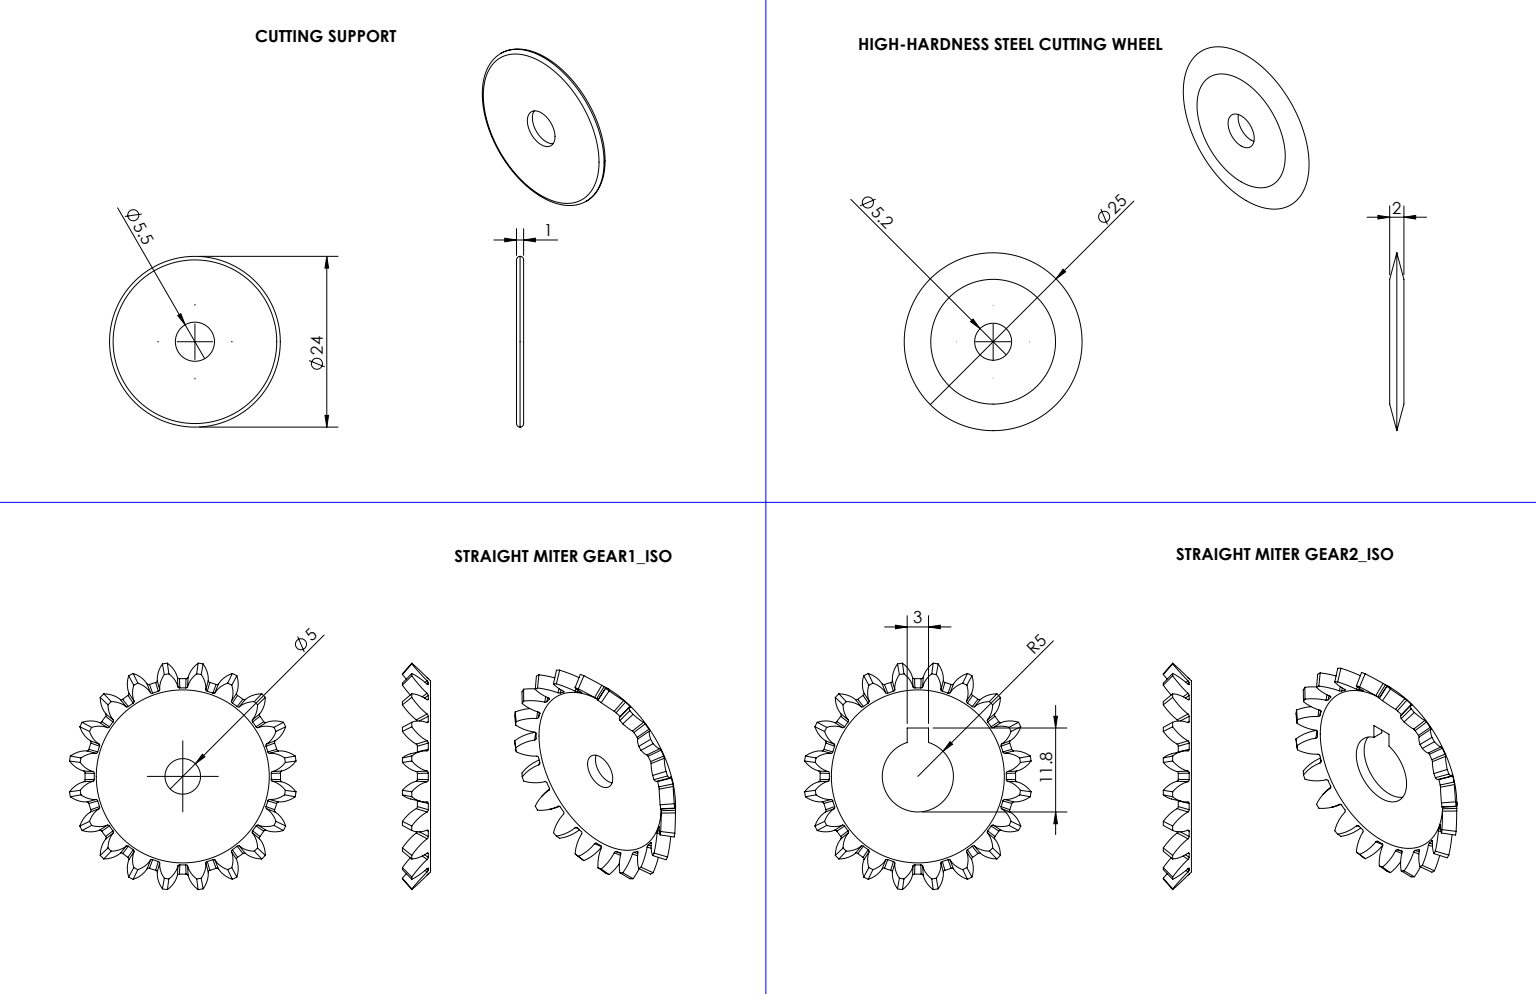
ISO-10303-21;
HEADER;
FILE_DESCRIPTION (('STEP AP214'),
    '1' );
FILE_NAME ('High-Hardness Steel Cutting Wheel.step',
    '2026-09-24T10:15:42',
    ( '' ),
    ( '' ),
    'SwSTEP 2.0',
    'SolidWorks 2026',
    '' );
FILE_SCHEMA (( 'AUTOMOTIVE_DESIGN' ));
ENDSEC;

DATA;
#92=FACE_BOUND ( 'NONE', #18498, .T. ) ;
#132=ORIENTED_EDGE ( 'NONE', *, *, #4909, .F. ) ;
#187=EDGE_LOOP ( 'NONE', ( #15081, #15539 ) ) ;
#218=SURFACE_SIDE_STYLE ('',( #5937 ) ) ;
#256=VERTEX_POINT ( 'NONE', #16289 ) ;
#279=ORIENTED_EDGE ( 'NONE', *, *, #2294, .T. ) ;
#396=MECHANICAL_DESIGN_GEOMETRIC_PRESENTATION_REPRESENTATION('',(#14763),#11087);
#455=PRODUCT_DEFINITION_CONTEXT ( 'detailed design', #9607, 'design' ) ;
#466=AXIS2_PLACEMENT_3D ( 'NONE', #18241, #2269, #18054 ) ;
#565=DIRECTION ( 'NONE',  ( -0.000000000000000000, 1.000000000000000000, -0.000000000000000000 ) ) ;
#601=ADVANCED_FACE ( 'NONE', ( #10334 ), #6040, .F. ) ;
#657=ORIENTED_EDGE ( 'NONE', *, *, #5467, .T. ) ;
#781=DIRECTION ( 'NONE',  ( 0.000000000000000000, -1.000000000000000000, 0.000000000000000000 ) ) ;
#795=EDGE_LOOP ( 'NONE', ( #16035, #279, #1272, #10918 ) ) ;
#851=ADVANCED_FACE ( 'NONE', ( #17477, #10119 ), #8682, .F. ) ;
#884=EDGE_LOOP ( 'NONE', ( #132, #11644, #15801, #8362 ) ) ;
#997=ORIENTED_EDGE ( 'NONE', *, *, #13718, .T. ) ;
#1073=EDGE_CURVE ( 'NONE', #15587, #15699, #16006, .T. ) ;
#1102=( GEOMETRIC_REPRESENTATION_CONTEXT ( 3 ) GLOBAL_UNCERTAINTY_ASSIGNED_CONTEXT ( ( #11702 ) ) GLOBAL_UNIT_ASSIGNED_CONTEXT ( ( #6049, #7298, #13114 ) ) REPRESENTATION_CONTEXT ( 'NONE', 'WORKASPACE' ) );
#1175=DIRECTION ( 'NONE',  ( 1.540743955509788340E-33, 1.000000000000000000, 2.533398541561209262E-17 ) ) ;
#1245=DIRECTION ( 'NONE',  ( 0.000000000000000000, 0.000000000000000000, 1.000000000000000000 ) ) ;
#1272=ORIENTED_EDGE ( 'NONE', *, *, #5435, .F. ) ;
#1327=CARTESIAN_POINT ( 'NONE',  ( 1.321128355694181398E-14, -7.013167318348350499, 25.01316734529530095 ) ) ;
#1414=PRODUCT ( 'High-Hardness Steel Cutting Wheel', 'High-Hardness Steel Cutting Wheel', '', ( #12280 ) ) ;
#1442=EDGE_LOOP ( 'NONE', ( #18668, #4195, #17241, #11960 ) ) ;
#1444=DIRECTION ( 'NONE',  ( 1.540743955509788340E-33, 1.000000000000000000, 2.533398541561209262E-17 ) ) ;
#1471=PRODUCT_DEFINITION ( 'UNKNOWN', '', #4710, #455 ) ;
#1479=EDGE_CURVE ( 'NONE', #15020, #256, #1980, .T. ) ;
#1562=AXIS2_PLACEMENT_3D ( 'NONE', #11635, #5692, #17463 ) ;
#1662=FACE_OUTER_BOUND ( 'NONE', #1442, .T. ) ;
#1671=VECTOR ( 'NONE', #15487, 1000.000000000000114 ) ;
#1803=ORIENTED_EDGE ( 'NONE', *, *, #4909, .T. ) ;
#1812=AXIS2_PLACEMENT_3D ( 'NONE', #15485, #781, #18442 ) ;
#1888=DIRECTION ( 'NONE',  ( -1.540743955509788340E-33, -1.000000000000000000, -2.533398541561209262E-17 ) ) ;
#1965=CARTESIAN_POINT ( 'NONE',  ( 1.451356985208877954E-14, -9.013167318348349610, 16.24521815286417947 ) ) ;
#1980=LINE ( 'NONE', #7820, #2247 ) ;
#2030=AXIS2_PLACEMENT_3D ( 'NONE', #15716, #11248, #17249 ) ;
#2049=AXIS2_PLACEMENT_3D ( 'NONE', #17593, #1444, #9087 ) ;
#2084=CONICAL_SURFACE ( 'NONE', #18539, 12.50000000000000355, 1.308996938995747428 ) ;
#2229=CARTESIAN_POINT ( 'NONE',  ( 1.321128355694181398E-14, -7.013167318348350499, 25.01316734529530095 ) ) ;
#2236=SURFACE_STYLE_FILL_AREA ( #9686 ) ;
#2247=VECTOR ( 'NONE', #6907, 1000.000000000000114 ) ;
#2269=DIRECTION ( 'NONE',  ( 1.540743955509788340E-33, 1.000000000000000000, 2.533398541561209262E-17 ) ) ;
#2294=EDGE_CURVE ( 'NONE', #12560, #15587, #14969, .T. ) ;
#2327=( NAMED_UNIT ( * ) PLANE_ANGLE_UNIT ( ) SI_UNIT ( $, .RADIAN. ) );
#2395=ORIENTED_EDGE ( 'NONE', *, *, #9782, .F. ) ;
#2464=EDGE_LOOP ( 'NONE', ( #11141, #1803, #13657, #3611 ) ) ;
#2532=DIRECTION ( 'NONE',  ( 0.000000000000000000, -0.2588190451025214611, -0.9659258262890679791 ) ) ;
#2742=DIRECTION ( 'NONE',  ( 0.000000000000000000, -2.533398541561209262E-17, 1.000000000000000000 ) ) ;
#2746=DIRECTION ( 'NONE',  ( 0.000000000000000000, -2.533398541561209262E-17, 1.000000000000000000 ) ) ;
#2869=DIRECTION ( 'NONE',  ( -0.000000000000000000, 1.000000000000000000, -0.000000000000000000 ) ) ;
#2879=VECTOR ( 'NONE', #2532, 1000.000000000000114 ) ;
#2951=CARTESIAN_POINT ( 'NONE',  ( 1.321128355694181398E-14, -8.013167318348353163, 12.51316734529529562 ) ) ;
#3058=PRESENTATION_STYLE_ASSIGNMENT (( #4615 ) ) ;
#3059=DIRECTION ( 'NONE',  ( 0.000000000000000000, 0.000000000000000000, 1.000000000000000000 ) ) ;
#3319=ORIENTED_EDGE ( 'NONE', *, *, #1073, .F. ) ;
#3343=VERTEX_POINT ( 'NONE', #18411 ) ;
#3495=EDGE_LOOP ( 'NONE', ( #9973, #17749 ) ) ;
#3611=ORIENTED_EDGE ( 'NONE', *, *, #1479, .F. ) ;
#3694=FACE_OUTER_BOUND ( 'NONE', #2464, .T. ) ;
#3833=LINE ( 'NONE', #9659, #1671 ) ;
#3858=( NAMED_UNIT ( * ) PLANE_ANGLE_UNIT ( ) SI_UNIT ( $, .RADIAN. ) );
#4195=ORIENTED_EDGE ( 'NONE', *, *, #5467, .F. ) ;
#4383=DIRECTION ( 'NONE',  ( 1.540743955509788340E-33, 1.000000000000000000, 2.533398541561209262E-17 ) ) ;
#4568=CIRCLE ( 'NONE', #13723, 12.50000000000000355 ) ;
#4615=SURFACE_STYLE_USAGE ( .BOTH. , #218 ) ;
#4710=PRODUCT_DEFINITION_FORMATION_WITH_SPECIFIED_SOURCE ( 'ANY', '', #1414, .NOT_KNOWN. ) ;
#4808=AXIS2_PLACEMENT_3D ( 'NONE', #7609, #12190, #7799 ) ;
#4909=EDGE_CURVE ( 'NONE', #18033, #5504, #7459, .T. ) ;
#5081=MECHANICAL_DESIGN_GEOMETRIC_PRESENTATION_REPRESENTATION('',(#16981),#1102);
#5195=SURFACE_SIDE_STYLE ('',( #2236 ) ) ;
#5244=EDGE_CURVE ( 'NONE', #12234, #3343, #18505, .T. ) ;
#5407=CARTESIAN_POINT ( 'NONE',  ( 1.104287921197080512E-14, -7.013167318348350499, 22.41316734529519650 ) ) ;
#5435=EDGE_CURVE ( 'NONE', #15699, #15587, #8163, .T. ) ;
#5467=EDGE_CURVE ( 'NONE', #3343, #12234, #10605, .T. ) ;
#5504=VERTEX_POINT ( 'NONE', #2951 ) ;
#5532=CARTESIAN_POINT ( 'NONE',  ( 1.104287921197080512E-14, -7.013167318348350499, 22.41316734529519650 ) ) ;
#5692=DIRECTION ( 'NONE',  ( -1.540743955509788340E-33, -1.000000000000000000, -2.533398541561209262E-17 ) ) ;
#5820=AXIS2_PLACEMENT_3D ( 'NONE', #15005, #7668, #11955 ) ;
#5937=SURFACE_STYLE_FILL_AREA ( #10440 ) ;
#5991=DIRECTION ( 'NONE',  ( 0.000000000000000000, 0.000000000000000000, 1.000000000000000000 ) ) ;
#6040=CYLINDRICAL_SURFACE ( 'NONE', #13619, 2.600000000000092015 ) ;
#6049=( LENGTH_UNIT ( ) NAMED_UNIT ( * ) SI_UNIT ( .MILLI., .METRE. ) );
#6129=CYLINDRICAL_SURFACE ( 'NONE', #5820, 2.600000000000092015 ) ;
#6330=DIRECTION ( 'NONE',  ( 0.000000000000000000, 0.000000000000000000, -1.000000000000000000 ) ) ;
#6514=ORIENTED_EDGE ( 'NONE', *, *, #17078, .F. ) ;
#6622=COLOUR_RGB ( '', 0.08235294, 0.09019608, 0.10196078) ;
#6708=ORIENTED_EDGE ( 'NONE', *, *, #18094, .T. ) ;
#6739=SHAPE_DEFINITION_REPRESENTATION ( #17767, #13515 ) ;
#6907=DIRECTION ( 'NONE',  ( 0.000000000000000000, 0.2588190451025206285, 0.9659258262890683122 ) ) ;
#6917=( LENGTH_UNIT ( ) NAMED_UNIT ( * ) SI_UNIT ( .MILLI., .METRE. ) );
#7015=DIRECTION ( 'NONE',  ( 0.000000000000000000, 0.000000000000000000, 1.000000000000000000 ) ) ;
#7174=DIRECTION ( 'NONE',  ( 1.540743955509788340E-33, 1.000000000000000000, 2.533398541561209262E-17 ) ) ;
#7248=DIRECTION ( 'NONE',  ( 0.000000000000000000, -1.000000000000000000, 0.000000000000000000 ) ) ;
#7249=CLOSED_SHELL ( 'NONE', ( #13576, #7332, #601, #8241, #851, #12848, #16673, #11406 ) ) ;
#7298=( NAMED_UNIT ( * ) PLANE_ANGLE_UNIT ( ) SI_UNIT ( $, .RADIAN. ) );
#7332=ADVANCED_FACE ( 'NONE', ( #15316 ), #12653, .T. ) ;
#7459=LINE ( 'NONE', #11846, #8088 ) ;
#7463=CARTESIAN_POINT ( 'NONE',  ( 1.321128355694181398E-14, -9.013167318348349610, 25.01316734529530095 ) ) ;
#7609=CARTESIAN_POINT ( 'NONE',  ( 1.321128355694181398E-14, -7.013167318348350499, 25.01316734529530095 ) ) ;
#7668=DIRECTION ( 'NONE',  ( -1.540743955509788340E-33, -1.000000000000000000, -2.533398541561209262E-17 ) ) ;
#7752=CONICAL_SURFACE ( 'NONE', #18696, 12.50000000000000355, 1.308996938995747428 ) ;
#7799=DIRECTION ( 'NONE',  ( 0.000000000000000000, 0.000000000000000000, -1.000000000000000000 ) ) ;
#7820=CARTESIAN_POINT ( 'NONE',  ( 1.321128355694181398E-14, -8.013167318348349610, 37.51316734529530805 ) ) ;
#7832=CARTESIAN_POINT ( 'NONE',  ( 1.321128355694181398E-14, -8.013167318348349610, 25.01316734529530095 ) ) ;
#7885=CARTESIAN_POINT ( 'NONE',  ( 1.136128737974912818E-14, -7.013167318348350499, 27.61316734529538053 ) ) ;
#7966=EDGE_CURVE ( 'NONE', #3343, #5504, #15454, .T. ) ;
#8062=DIRECTION ( 'NONE',  ( 0.000000000000000000, 0.000000000000000000, 1.000000000000000000 ) ) ;
#8083=CARTESIAN_POINT ( 'NONE',  ( 1.451356985208878270E-14, -7.013167318348350499, 33.78111653772643308 ) ) ;
#8088=VECTOR ( 'NONE', #17577, 1000.000000000000114 ) ;
#8163=CIRCLE ( 'NONE', #18823, 2.600000000000092015 ) ;
#8241=ADVANCED_FACE ( 'NONE', ( #8593, #92 ), #17685, .T. ) ;
#8265=( LENGTH_UNIT ( ) NAMED_UNIT ( * ) SI_UNIT ( .MILLI., .METRE. ) );
#8362=ORIENTED_EDGE ( 'NONE', *, *, #17496, .T. ) ;
#8375=EDGE_LOOP ( 'NONE', ( #16741, #10834, #997, #3319 ) ) ;
#8466=DIRECTION ( 'NONE',  ( -1.540743955509788340E-33, -1.000000000000000000, -2.533398541561209262E-17 ) ) ;
#8516=CARTESIAN_POINT ( 'NONE',  ( 1.104287921197080512E-14, -9.013167318348349610, 25.01316734529528674 ) ) ;
#8593=FACE_OUTER_BOUND ( 'NONE', #13210, .T. ) ;
#8629=APPLICATION_CONTEXT ( 'automotive_design' ) ;
#8659=ORIENTED_EDGE ( 'NONE', *, *, #7966, .F. ) ;
#8682=PLANE ( 'NONE',  #14026 ) ;
#9004=ADVANCED_BREP_SHAPE_REPRESENTATION ( '', ( #10342, #2030 ), #13001 ) ;
#9007=SHAPE_REPRESENTATION_RELATIONSHIP ( 'NONE' , 'NONE' ,  #13515, #9004 ) ;
#9087=DIRECTION ( 'NONE',  ( 0.000000000000000000, 0.000000000000000000, 1.000000000000000000 ) ) ;
#9132=CARTESIAN_POINT ( 'NONE',  ( 1.321128355694181398E-14, -9.013167318348349610, 33.78111653772642597 ) ) ;
#9178=FACE_OUTER_BOUND ( 'NONE', #8375, .T. ) ;
#9607=APPLICATION_CONTEXT ( 'automotive_design' ) ;
#9659=CARTESIAN_POINT ( 'NONE',  ( 1.428504764830155575E-14, -7.013167318348350499, 33.78111653772643308 ) ) ;
#9686=FILL_AREA_STYLE ('',( #15865 ) ) ;
#9782=EDGE_CURVE ( 'NONE', #12560, #18215, #17894, .T. ) ;
#9926=DIRECTION ( 'NONE',  ( 1.540743955509788340E-33, 1.000000000000000000, 2.533398541561209262E-17 ) ) ;
#9973=ORIENTED_EDGE ( 'NONE', *, *, #17326, .T. ) ;
#10034=CIRCLE ( 'NONE', #1812, 12.50000000000000355 ) ;
#10119=FACE_BOUND ( 'NONE', #187, .T. ) ;
#10334=FACE_OUTER_BOUND ( 'NONE', #795, .T. ) ;
#10342=MANIFOLD_SOLID_BREP ( 'Chamfer2', #7249 ) ;
#10368=UNCERTAINTY_MEASURE_WITH_UNIT (LENGTH_MEASURE( 1.000000000000000082E-05 ), #6917, 'distance_accuracy_value', 'NONE');
#10440=FILL_AREA_STYLE ('',( #17417 ) ) ;
#10531=ORIENTED_EDGE ( 'NONE', *, *, #11357, .F. ) ;
#10605=CIRCLE ( 'NONE', #2049, 8.767949192431130356 ) ;
#10746=DIRECTION ( 'NONE',  ( 0.000000000000000000, 0.000000000000000000, -1.000000000000000000 ) ) ;
#10834=ORIENTED_EDGE ( 'NONE', *, *, #9782, .T. ) ;
#10918=ORIENTED_EDGE ( 'NONE', *, *, #13718, .F. ) ;
#10988=AXIS2_PLACEMENT_3D ( 'NONE', #7463, #17878, #14905 ) ;
#11087=( GEOMETRIC_REPRESENTATION_CONTEXT ( 3 ) GLOBAL_UNCERTAINTY_ASSIGNED_CONTEXT ( ( #12635 ) ) GLOBAL_UNIT_ASSIGNED_CONTEXT ( ( #8265, #2327, #13889 ) ) REPRESENTATION_CONTEXT ( 'NONE', 'WORKASPACE' ) );
#11141=ORIENTED_EDGE ( 'NONE', *, *, #12931, .F. ) ;
#11248=DIRECTION ( 'NONE',  ( 0.000000000000000000, 0.000000000000000000, 1.000000000000000000 ) ) ;
#11263=CARTESIAN_POINT ( 'NONE',  ( 1.321128355694181398E-14, -7.013167318348350499, 16.24521815286417237 ) ) ;
#11357=EDGE_CURVE ( 'NONE', #18215, #12560, #15963, .T. ) ;
#11406=ADVANCED_FACE ( 'NONE', ( #13206 ), #7752, .T. ) ;
#11475=CARTESIAN_POINT ( 'NONE',  ( 1.104287921197080512E-14, -7.013167318348350499, 25.01316734529528674 ) ) ;
#11572=SURFACE_STYLE_USAGE ( .BOTH. , #5195 ) ;
#11600=ORIENTED_EDGE ( 'NONE', *, *, #5244, .T. ) ;
#11635=CARTESIAN_POINT ( 'NONE',  ( 1.321128355694181398E-14, -9.013167318348349610, 25.01316734529530095 ) ) ;
#11644=ORIENTED_EDGE ( 'NONE', *, *, #17326, .F. ) ;
#11702=UNCERTAINTY_MEASURE_WITH_UNIT (LENGTH_MEASURE( 1.000000000000000082E-05 ), #6049, 'distance_accuracy_value', 'NONE');
#11741=VECTOR ( 'NONE', #1888, 1000.000000000000000 ) ;
#11846=CARTESIAN_POINT ( 'NONE',  ( 1.474209205587600649E-14, -8.013167318348349610, 12.51316734529529562 ) ) ;
#11955=DIRECTION ( 'NONE',  ( 0.000000000000000000, 0.000000000000000000, -1.000000000000000000 ) ) ;
#11960=ORIENTED_EDGE ( 'NONE', *, *, #17496, .F. ) ;
#12190=DIRECTION ( 'NONE',  ( 0.000000000000000000, -1.000000000000000000, 0.000000000000000000 ) ) ;
#12234=VERTEX_POINT ( 'NONE', #8083 ) ;
#12280=PRODUCT_CONTEXT ( 'NONE', #8629, 'mechanical' ) ;
#12393=DIRECTION ( 'NONE',  ( 0.000000000000000000, 0.000000000000000000, 1.000000000000000000 ) ) ;
#12560=VERTEX_POINT ( 'NONE', #7885 ) ;
#12635=UNCERTAINTY_MEASURE_WITH_UNIT (LENGTH_MEASURE( 1.000000000000000082E-05 ), #8265, 'distance_accuracy_value', 'NONE');
#12653=CONICAL_SURFACE ( 'NONE', #13573, 8.767949192431130356, 1.308996938995746318 ) ;
#12793=CARTESIAN_POINT ( 'NONE',  ( 1.321128355694181398E-14, -9.013167318348349610, 25.01316734529530095 ) ) ;
#12848=ADVANCED_FACE ( 'NONE', ( #9178 ), #6129, .F. ) ;
#12931=EDGE_CURVE ( 'NONE', #18033, #15020, #15900, .T. ) ;
#13001=( GEOMETRIC_REPRESENTATION_CONTEXT ( 3 ) GLOBAL_UNCERTAINTY_ASSIGNED_CONTEXT ( ( #10368 ) ) GLOBAL_UNIT_ASSIGNED_CONTEXT ( ( #6917, #3858, #18565 ) ) REPRESENTATION_CONTEXT ( 'NONE', 'WORKASPACE' ) );
#13018=CARTESIAN_POINT ( 'NONE',  ( 1.321128355694181398E-14, -8.013167318348349610, 25.01316734529530095 ) ) ;
#13114=( NAMED_UNIT ( * ) SI_UNIT ( $, .STERADIAN. ) SOLID_ANGLE_UNIT ( ) );
#13206=FACE_OUTER_BOUND ( 'NONE', #884, .T. ) ;
#13210=EDGE_LOOP ( 'NONE', ( #657, #11600 ) ) ;
#13353=CARTESIAN_POINT ( 'NONE',  ( 1.321128355694181398E-14, -8.013167318348353163, 25.01316734529530095 ) ) ;
#13515=SHAPE_REPRESENTATION ( 'High-Hardness Steel Cutting Wheel', ( #2030 ), #13001 ) ;
#13573=AXIS2_PLACEMENT_3D ( 'NONE', #2229, #13609, #10746 ) ;
#13576=ADVANCED_FACE ( 'NONE', ( #3694 ), #2084, .T. ) ;
#13609=DIRECTION ( 'NONE',  ( 0.000000000000000000, -1.000000000000000000, 0.000000000000000000 ) ) ;
#13619=AXIS2_PLACEMENT_3D ( 'NONE', #16365, #16265, #6330 ) ;
#13657=ORIENTED_EDGE ( 'NONE', *, *, #17078, .T. ) ;
#13718=EDGE_CURVE ( 'NONE', #18215, #15699, #14381, .T. ) ;
#13723=AXIS2_PLACEMENT_3D ( 'NONE', #13353, #7248, #5991 ) ;
#13889=( NAMED_UNIT ( * ) SI_UNIT ( $, .STERADIAN. ) SOLID_ANGLE_UNIT ( ) );
#13970=CARTESIAN_POINT ( 'NONE',  ( 1.136128737974912818E-14, -9.013167318348349610, 27.61316734529538053 ) ) ;
#14026=AXIS2_PLACEMENT_3D ( 'NONE', #12793, #4383, #2742 ) ;
#14058=DIRECTION ( 'NONE',  ( 0.000000000000000000, 0.000000000000000000, 1.000000000000000000 ) ) ;
#14274=CARTESIAN_POINT ( 'NONE',  ( 1.104287921197080512E-14, -7.013167318348350499, 25.01316734529528674 ) ) ;
#14341=DIRECTION ( 'NONE',  ( 1.540743955509788340E-33, 1.000000000000000000, 2.533398541561209262E-17 ) ) ;
#14381=LINE ( 'NONE', #5407, #16116 ) ;
#14504=AXIS2_PLACEMENT_3D ( 'NONE', #11475, #7174, #14058 ) ;
#14763=STYLED_ITEM ( 'NONE', ( #17292 ), #10342 ) ;
#14905=DIRECTION ( 'NONE',  ( 0.000000000000000000, 0.000000000000000000, 1.000000000000000000 ) ) ;
#14969=LINE ( 'NONE', #17849, #11741 ) ;
#15005=CARTESIAN_POINT ( 'NONE',  ( 1.104287921197080512E-14, -7.013167318348350499, 25.01316734529528674 ) ) ;
#15020=VERTEX_POINT ( 'NONE', #9132 ) ;
#15081=ORIENTED_EDGE ( 'NONE', *, *, #5435, .T. ) ;
#15224=DIRECTION ( 'NONE',  ( 1.540743955509788340E-33, 1.000000000000000000, 2.533398541561209262E-17 ) ) ;
#15307=CARTESIAN_POINT ( 'NONE',  ( 1.321128355694181398E-14, -7.013167318348350499, 25.01316734529530095 ) ) ;
#15316=FACE_OUTER_BOUND ( 'NONE', #16211, .T. ) ;
#15454=LINE ( 'NONE', #11263, #2879 ) ;
#15485=CARTESIAN_POINT ( 'NONE',  ( 1.321128355694181398E-14, -8.013167318348353163, 25.01316734529530095 ) ) ;
#15487=DIRECTION ( 'NONE',  ( 1.182917971378669349E-16, -0.2588190451025214611, 0.9659258262890679791 ) ) ;
#15539=ORIENTED_EDGE ( 'NONE', *, *, #1073, .T. ) ;
#15587=VERTEX_POINT ( 'NONE', #13970 ) ;
#15699=VERTEX_POINT ( 'NONE', #16160 ) ;
#15716=CARTESIAN_POINT ( 'NONE',  ( 0.000000000000000000, 0.000000000000000000, 0.000000000000000000 ) ) ;
#15801=ORIENTED_EDGE ( 'NONE', *, *, #1479, .T. ) ;
#15865=FILL_AREA_STYLE_COLOUR ( '', #16873 ) ;
#15900=CIRCLE ( 'NONE', #1562, 8.767949192431123251 ) ;
#15963=CIRCLE ( 'NONE', #18108, 2.600000000000092015 ) ;
#16006=CIRCLE ( 'NONE', #466, 2.600000000000092015 ) ;
#16035=ORIENTED_EDGE ( 'NONE', *, *, #11357, .T. ) ;
#16116=VECTOR ( 'NONE', #8466, 1000.000000000000000 ) ;
#16160=CARTESIAN_POINT ( 'NONE',  ( 1.104287921197080512E-14, -9.013167318348349610, 22.41316734529519650 ) ) ;
#16211=EDGE_LOOP ( 'NONE', ( #17374, #6708, #6514, #8659 ) ) ;
#16265=DIRECTION ( 'NONE',  ( -1.540743955509788340E-33, -1.000000000000000000, -2.533398541561209262E-17 ) ) ;
#16289=CARTESIAN_POINT ( 'NONE',  ( 1.474209205587600965E-14, -8.013167318348353163, 37.51316734529530805 ) ) ;
#16365=CARTESIAN_POINT ( 'NONE',  ( 1.104287921197080512E-14, -7.013167318348350499, 25.01316734529528674 ) ) ;
#16673=ADVANCED_FACE ( 'NONE', ( #1662 ), #18826, .T. ) ;
#16697=AXIS2_PLACEMENT_3D ( 'NONE', #15307, #15224, #8062 ) ;
#16741=ORIENTED_EDGE ( 'NONE', *, *, #2294, .F. ) ;
#16873=COLOUR_RGB ( '', 0.08235294, 0.09019608, 0.10196078) ;
#16981=STYLED_ITEM ( 'NONE', ( #3058 ), #9004 ) ;
#17078=EDGE_CURVE ( 'NONE', #5504, #256, #10034, .T. ) ;
#17241=ORIENTED_EDGE ( 'NONE', *, *, #7966, .T. ) ;
#17249=DIRECTION ( 'NONE',  ( 1.000000000000000000, 0.000000000000000000, 0.000000000000000000 ) ) ;
#17292=PRESENTATION_STYLE_ASSIGNMENT (( #11572 ) ) ;
#17326=EDGE_CURVE ( 'NONE', #15020, #18033, #17697, .T. ) ;
#17374=ORIENTED_EDGE ( 'NONE', *, *, #5244, .F. ) ;
#17417=FILL_AREA_STYLE_COLOUR ( '', #6622 ) ;
#17463=DIRECTION ( 'NONE',  ( 0.000000000000000000, 0.000000000000000000, 1.000000000000000000 ) ) ;
#17477=FACE_OUTER_BOUND ( 'NONE', #3495, .T. ) ;
#17496=EDGE_CURVE ( 'NONE', #256, #5504, #4568, .T. ) ;
#17577=DIRECTION ( 'NONE',  ( 1.182917971378669595E-16, 0.2588190451025206285, -0.9659258262890683122 ) ) ;
#17593=CARTESIAN_POINT ( 'NONE',  ( 1.321128355694181398E-14, -7.013167318348350499, 25.01316734529530095 ) ) ;
#17685=PLANE ( 'NONE',  #17870 ) ;
#17697=CIRCLE ( 'NONE', #10988, 8.767949192431123251 ) ;
#17749=ORIENTED_EDGE ( 'NONE', *, *, #12931, .T. ) ;
#17767=PRODUCT_DEFINITION_SHAPE ( 'NONE', 'NONE',  #1471 ) ;
#17849=CARTESIAN_POINT ( 'NONE',  ( 1.136128737974912818E-14, -7.013167318348350499, 27.61316734529538053 ) ) ;
#17870=AXIS2_PLACEMENT_3D ( 'NONE', #1327, #9926, #2746 ) ;
#17878=DIRECTION ( 'NONE',  ( -1.540743955509788340E-33, -1.000000000000000000, -2.533398541561209262E-17 ) ) ;
#17894=CIRCLE ( 'NONE', #14504, 2.600000000000092015 ) ;
#18033=VERTEX_POINT ( 'NONE', #1965 ) ;
#18054=DIRECTION ( 'NONE',  ( 0.000000000000000000, 0.000000000000000000, 1.000000000000000000 ) ) ;
#18094=EDGE_CURVE ( 'NONE', #12234, #256, #3833, .T. ) ;
#18108=AXIS2_PLACEMENT_3D ( 'NONE', #14274, #1175, #7015 ) ;
#18215=VERTEX_POINT ( 'NONE', #5532 ) ;
#18241=CARTESIAN_POINT ( 'NONE',  ( 1.104287921197080512E-14, -9.013167318348349610, 25.01316734529528674 ) ) ;
#18411=CARTESIAN_POINT ( 'NONE',  ( 1.321128355694181398E-14, -7.013167318348350499, 16.24521815286417237 ) ) ;
#18442=DIRECTION ( 'NONE',  ( 0.000000000000000000, 0.000000000000000000, 1.000000000000000000 ) ) ;
#18498=EDGE_LOOP ( 'NONE', ( #10531, #2395 ) ) ;
#18505=CIRCLE ( 'NONE', #16697, 8.767949192431130356 ) ;
#18539=AXIS2_PLACEMENT_3D ( 'NONE', #7832, #565, #12393 ) ;
#18565=( NAMED_UNIT ( * ) SI_UNIT ( $, .STERADIAN. ) SOLID_ANGLE_UNIT ( ) );
#18668=ORIENTED_EDGE ( 'NONE', *, *, #18094, .F. ) ;
#18696=AXIS2_PLACEMENT_3D ( 'NONE', #13018, #2869, #3059 ) ;
#18823=AXIS2_PLACEMENT_3D ( 'NONE', #8516, #14341, #1245 ) ;
#18826=CONICAL_SURFACE ( 'NONE', #4808, 8.767949192431130356, 1.308996938995746318 ) ;
ENDSEC;
END-ISO-10303-21;
